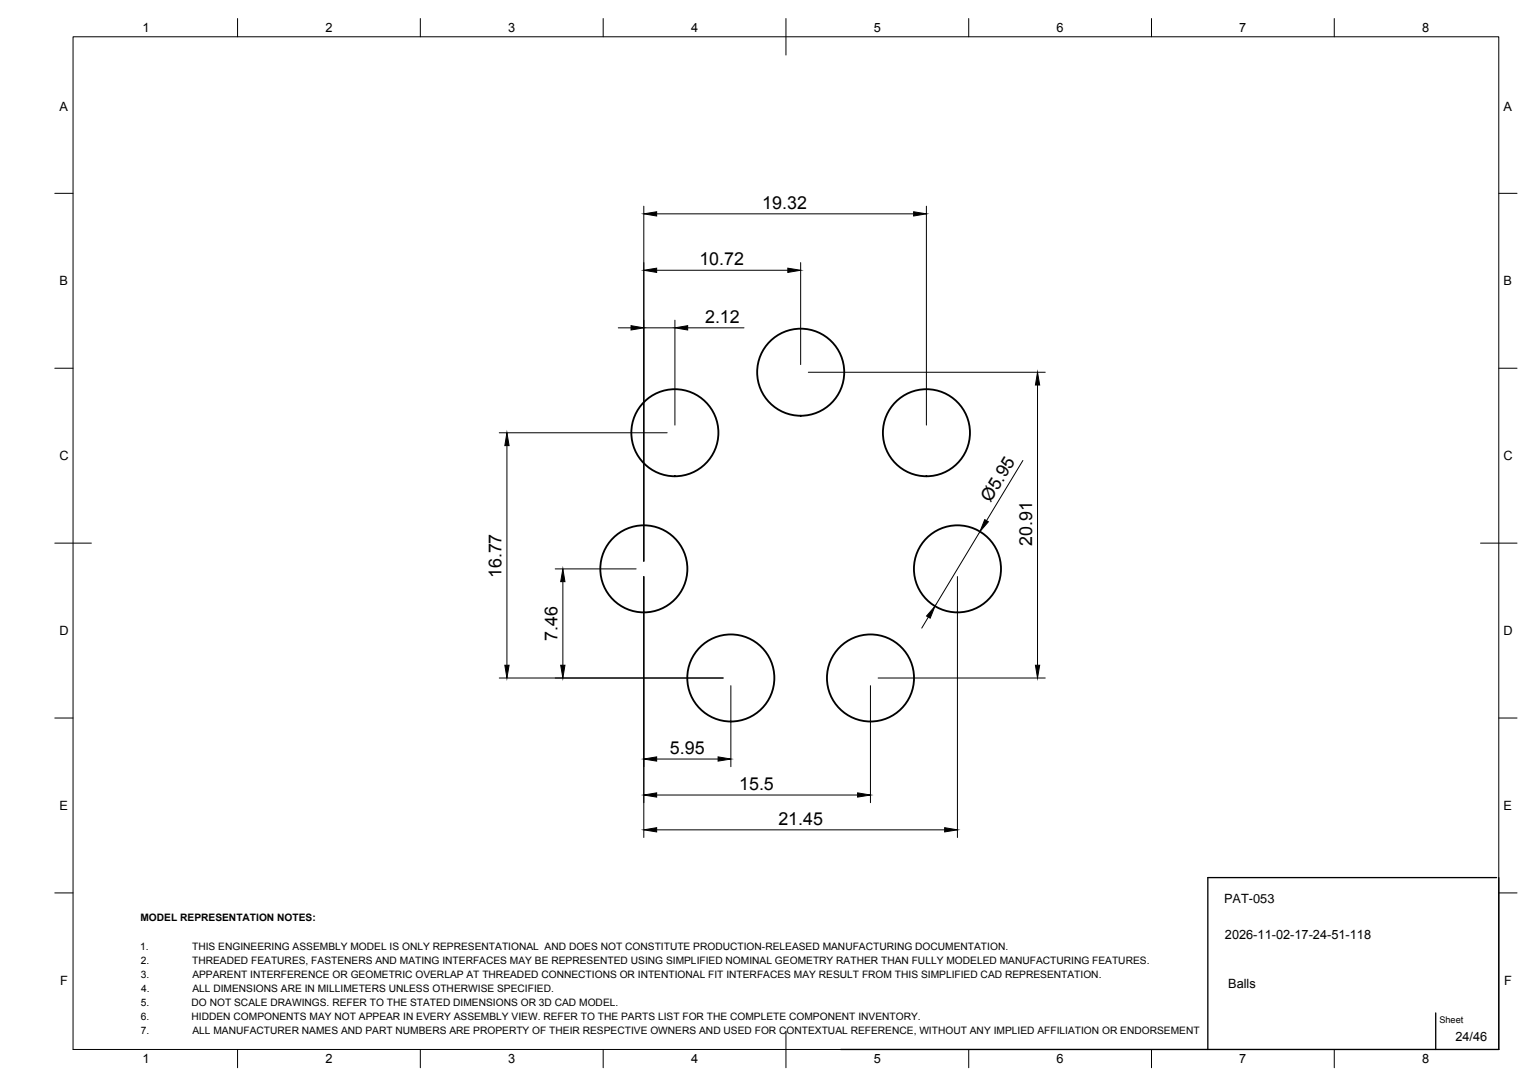
ISO-10303-21;
HEADER;
/* Generated by software containing ST-Developer
 * from STEP Tools, Inc. (www.steptools.com) 
 */

FILE_DESCRIPTION(
/* description */ ('Hand-operated arbor press'),
/* implementation_level */ '2;1');

FILE_NAME(
/* name */ 'Balls.step',
/* time_stamp */ '2026-10-28T03:25:25-07:00',
/* author */ (''),
/* organization */ (''),
/* preprocessor_version */ 'ST-DEVELOPER v20.2',
/* originating_system */ 'Autodesk Translation Framework v15.17.0.0',
/* authorisation */ '');

FILE_SCHEMA (('AUTOMOTIVE_DESIGN { 1 0 10303 214 3 1 1 }'));
ENDSEC;

DATA;
#10=MECHANICAL_DESIGN_GEOMETRIC_PRESENTATION_REPRESENTATION('',(#604,#605,#606,#607,#608,#609,#610),#32751);
#457=SPHERICAL_SURFACE('',#13456,0.29765);
#458=SPHERICAL_SURFACE('',#13458,0.29765);
#459=SPHERICAL_SURFACE('',#13460,0.29765);
#460=SPHERICAL_SURFACE('',#13462,0.29765);
#461=SPHERICAL_SURFACE('',#13464,0.29765);
#462=SPHERICAL_SURFACE('',#13466,0.29765);
#463=SPHERICAL_SURFACE('',#13468,0.29765);
#520=SHAPE_REPRESENTATION_RELATIONSHIP('SRR','None',#32950,#562);
#562=ADVANCED_BREP_SHAPE_REPRESENTATION('',(#652,#653,#654,#655,#656,#657,
#658),#32724);
#604=STYLED_ITEM('',(#33242),#652);
#605=STYLED_ITEM('',(#33242),#653);
#606=STYLED_ITEM('',(#33242),#654);
#607=STYLED_ITEM('',(#33242),#655);
#608=STYLED_ITEM('',(#33242),#656);
#609=STYLED_ITEM('',(#33242),#657);
#610=STYLED_ITEM('',(#33242),#658);
#652=MANIFOLD_SOLID_BREP('Body1',#12502);
#653=MANIFOLD_SOLID_BREP('Body2',#12503);
#654=MANIFOLD_SOLID_BREP('Body3',#12504);
#655=MANIFOLD_SOLID_BREP('Body4',#12505);
#656=MANIFOLD_SOLID_BREP('Body5',#12506);
#657=MANIFOLD_SOLID_BREP('Body6',#12507);
#658=MANIFOLD_SOLID_BREP('Body7',#12508);
#1528=FACE_OUTER_BOUND('',#2335,.T.);
#1529=FACE_OUTER_BOUND('',#2336,.T.);
#1530=FACE_OUTER_BOUND('',#2337,.T.);
#1531=FACE_OUTER_BOUND('',#2338,.T.);
#1532=FACE_OUTER_BOUND('',#2339,.T.);
#1533=FACE_OUTER_BOUND('',#2340,.T.);
#1534=FACE_OUTER_BOUND('',#2341,.T.);
#2335=EDGE_LOOP('',(#9406,#9407));
#2336=EDGE_LOOP('',(#9408,#9409));
#2337=EDGE_LOOP('',(#9410,#9411));
#2338=EDGE_LOOP('',(#9412,#9413));
#2339=EDGE_LOOP('',(#9414,#9415));
#2340=EDGE_LOOP('',(#9416,#9417));
#2341=EDGE_LOOP('',(#9418,#9419));
#5366=CIRCLE('',#13457,0.29765);
#5367=CIRCLE('',#13459,0.29765);
#5368=CIRCLE('',#13461,0.29765);
#5369=CIRCLE('',#13463,0.29765);
#5370=CIRCLE('',#13465,0.29765);
#5371=CIRCLE('',#13467,0.29765);
#5372=CIRCLE('',#13469,0.29765);
#5914=VERTEX_POINT('',#18795);
#5915=VERTEX_POINT('',#18796);
#5916=VERTEX_POINT('',#18799);
#5917=VERTEX_POINT('',#18800);
#5918=VERTEX_POINT('',#18803);
#5919=VERTEX_POINT('',#18804);
#5920=VERTEX_POINT('',#18807);
#5921=VERTEX_POINT('',#18808);
#5922=VERTEX_POINT('',#18811);
#5923=VERTEX_POINT('',#18812);
#5924=VERTEX_POINT('',#18815);
#5925=VERTEX_POINT('',#18816);
#5926=VERTEX_POINT('',#18819);
#5927=VERTEX_POINT('',#18820);
#7206=EDGE_CURVE('',#5914,#5915,#5366,.T.);
#7207=EDGE_CURVE('',#5916,#5917,#5367,.T.);
#7208=EDGE_CURVE('',#5918,#5919,#5368,.T.);
#7209=EDGE_CURVE('',#5920,#5921,#5369,.T.);
#7210=EDGE_CURVE('',#5922,#5923,#5370,.T.);
#7211=EDGE_CURVE('',#5924,#5925,#5371,.T.);
#7212=EDGE_CURVE('',#5926,#5927,#5372,.T.);
#9406=ORIENTED_EDGE('',*,*,#7206,.T.);
#9407=ORIENTED_EDGE('',*,*,#7206,.F.);
#9408=ORIENTED_EDGE('',*,*,#7207,.T.);
#9409=ORIENTED_EDGE('',*,*,#7207,.F.);
#9410=ORIENTED_EDGE('',*,*,#7208,.T.);
#9411=ORIENTED_EDGE('',*,*,#7208,.F.);
#9412=ORIENTED_EDGE('',*,*,#7209,.T.);
#9413=ORIENTED_EDGE('',*,*,#7209,.F.);
#9414=ORIENTED_EDGE('',*,*,#7210,.T.);
#9415=ORIENTED_EDGE('',*,*,#7210,.F.);
#9416=ORIENTED_EDGE('',*,*,#7211,.T.);
#9417=ORIENTED_EDGE('',*,*,#7211,.F.);
#9418=ORIENTED_EDGE('',*,*,#7212,.T.);
#9419=ORIENTED_EDGE('',*,*,#7212,.F.);
#12037=ADVANCED_FACE('',(#1528),#457,.T.);
#12038=ADVANCED_FACE('',(#1529),#458,.T.);
#12039=ADVANCED_FACE('',(#1530),#459,.T.);
#12040=ADVANCED_FACE('',(#1531),#460,.T.);
#12041=ADVANCED_FACE('',(#1532),#461,.T.);
#12042=ADVANCED_FACE('',(#1533),#462,.T.);
#12043=ADVANCED_FACE('',(#1534),#463,.T.);
#12502=CLOSED_SHELL('',(#12037));
#12503=CLOSED_SHELL('',(#12038));
#12504=CLOSED_SHELL('',(#12039));
#12505=CLOSED_SHELL('',(#12040));
#12506=CLOSED_SHELL('',(#12041));
#12507=CLOSED_SHELL('',(#12042));
#12508=CLOSED_SHELL('',(#12043));
#13455=AXIS2_PLACEMENT_3D('',#18793,#15408,#15409);
#13456=AXIS2_PLACEMENT_3D('',#18794,#15410,#15411);
#13457=AXIS2_PLACEMENT_3D('',#18797,#15412,#15413);
#13458=AXIS2_PLACEMENT_3D('',#18798,#15414,#15415);
#13459=AXIS2_PLACEMENT_3D('',#18801,#15416,#15417);
#13460=AXIS2_PLACEMENT_3D('',#18802,#15418,#15419);
#13461=AXIS2_PLACEMENT_3D('',#18805,#15420,#15421);
#13462=AXIS2_PLACEMENT_3D('',#18806,#15422,#15423);
#13463=AXIS2_PLACEMENT_3D('',#18809,#15424,#15425);
#13464=AXIS2_PLACEMENT_3D('',#18810,#15426,#15427);
#13465=AXIS2_PLACEMENT_3D('',#18813,#15428,#15429);
#13466=AXIS2_PLACEMENT_3D('',#18814,#15430,#15431);
#13467=AXIS2_PLACEMENT_3D('',#18817,#15432,#15433);
#13468=AXIS2_PLACEMENT_3D('',#18818,#15434,#15435);
#13469=AXIS2_PLACEMENT_3D('',#18821,#15436,#15437);
#15408=DIRECTION('axis',(0.,0.,1.));
#15409=DIRECTION('refdir',(1.,0.,0.));
#15410=DIRECTION('center_axis',(0.,0.,1.));
#15411=DIRECTION('ref_axis',(1.,0.,0.));
#15412=DIRECTION('center_axis',(1.22464679914735E-16,-1.,0.));
#15413=DIRECTION('ref_axis',(-1.,-1.22464679914735E-16,0.));
#15414=DIRECTION('center_axis',(0.78183148246803,0.,0.623489801858733));
#15415=DIRECTION('ref_axis',(0.623489801858734,0.,-0.78183148246803));
#15416=DIRECTION('center_axis',(7.63554790147315E-17,-1.,-9.57467422477103E-17));
#15417=DIRECTION('ref_axis',(-0.623489801858734,-1.22464679914735E-16,0.78183148246803));
#15418=DIRECTION('center_axis',(0.974927912181824,0.,-0.222520933956314));
#15419=DIRECTION('ref_axis',(-0.222520933956314,0.,-0.974927912181824));
#15420=DIRECTION('center_axis',(-2.7250954951288E-17,-1.,-1.19394234705288E-16));
#15421=DIRECTION('ref_axis',(0.222520933956314,-1.22464679914735E-16,0.974927912181824));
#15422=DIRECTION('center_axis',(0.433883739117558,0.,-0.900968867902419));
#15423=DIRECTION('ref_axis',(-0.900968867902419,0.,-0.433883739117558));
#15424=DIRECTION('center_axis',(-1.10336864020811E-16,-1.,-5.31354332312403E-17));
#15425=DIRECTION('ref_axis',(0.900968867902419,-1.22464679914735E-16,0.433883739117558));
#15426=DIRECTION('center_axis',(-0.433883739117558,0.,-0.900968867902419));
#15427=DIRECTION('ref_axis',(-0.900968867902419,0.,0.433883739117558));
#15428=DIRECTION('center_axis',(-1.10336864020811E-16,-1.,5.31354332312403E-17));
#15429=DIRECTION('ref_axis',(0.900968867902419,-1.22464679914735E-16,-0.433883739117558));
#15430=DIRECTION('center_axis',(-0.974927912181824,0.,-0.222520933956314));
#15431=DIRECTION('ref_axis',(-0.222520933956315,0.,0.974927912181824));
#15432=DIRECTION('center_axis',(-2.7250954951288E-17,-1.,1.19394234705288E-16));
#15433=DIRECTION('ref_axis',(0.222520933956315,-1.22464679914735E-16,-0.974927912181824));
#15434=DIRECTION('center_axis',(-0.78183148246803,0.,0.623489801858734));
#15435=DIRECTION('ref_axis',(0.623489801858733,0.,0.78183148246803));
#15436=DIRECTION('center_axis',(7.63554790147315E-17,-1.,9.57467422477103E-17));
#15437=DIRECTION('ref_axis',(-0.623489801858733,-1.22464679914735E-16,-0.78183148246803));
#18793=CARTESIAN_POINT('',(0.,0.,0.));
#18794=CARTESIAN_POINT('Origin',(1.1,0.,0.));
#18795=CARTESIAN_POINT('',(1.1,-2.23201749654651E-33,0.29765));
#18796=CARTESIAN_POINT('',(1.1,-2.23201749654651E-33,-0.29765));
#18797=CARTESIAN_POINT('Origin',(1.1,0.,0.));
#18798=CARTESIAN_POINT('Origin',(0.685838782044607,0.,-0.860014630714833));
#18799=CARTESIAN_POINT('',(0.918550922801216,-5.31350540756609E-33,-0.674432891191581));
#18800=CARTESIAN_POINT('',(0.453126641287998,8.49470414473068E-34,-1.04559637023808));
#18801=CARTESIAN_POINT('Origin',(0.685838782044607,0.,-0.860014630714833));
#18802=CARTESIAN_POINT('Origin',(-0.244773027351946,0.,-1.07242070340001));
#18803=CARTESIAN_POINT('',(0.0454142657089739,-2.23201749654651E-33,-1.1386540593921));
#18804=CARTESIAN_POINT('',(-0.534960320412865,-2.23201749654651E-33,-1.00618734740791));
#18805=CARTESIAN_POINT('Origin',(-0.244773027351946,0.,-1.07242070340001));
#18806=CARTESIAN_POINT('Origin',(-0.991065754692661,0.,-0.477272113029314));
#18807=CARTESIAN_POINT('',(-0.86192025974432,8.49470414473067E-34,-0.745445496560469));
#18808=CARTESIAN_POINT('',(-1.120211249641,-5.31350540756609E-33,-0.209098729498159));
#18809=CARTESIAN_POINT('Origin',(-0.991065754692661,0.,-0.477272113029314));
#18810=CARTESIAN_POINT('Origin',(-0.991065754692661,0.,0.477272113029314));
#18811=CARTESIAN_POINT('',(-1.120211249641,-2.23201749654651E-33,0.209098729498159));
#18812=CARTESIAN_POINT('',(-0.86192025974432,-2.23201749654651E-33,0.745445496560469));
#18813=CARTESIAN_POINT('Origin',(-0.991065754692661,0.,0.477272113029314));
#18814=CARTESIAN_POINT('Origin',(-0.244773027351946,0.,1.07242070340001));
#18815=CARTESIAN_POINT('',(-0.534960320412866,-2.23201749654651E-33,1.00618734740791));
#18816=CARTESIAN_POINT('',(0.0454142657089737,-2.23201749654651E-33,1.1386540593921));
#18817=CARTESIAN_POINT('Origin',(-0.244773027351946,0.,1.07242070340001));
#18818=CARTESIAN_POINT('Origin',(0.685838782044607,0.,0.860014630714833));
#18819=CARTESIAN_POINT('',(0.453126641287998,-2.23201749654651E-33,1.04559637023808));
#18820=CARTESIAN_POINT('',(0.918550922801216,-2.23201749654651E-33,0.674432891191581));
#18821=CARTESIAN_POINT('Origin',(0.685838782044607,0.,0.860014630714833));
#32675=UNCERTAINTY_MEASURE_WITH_UNIT(LENGTH_MEASURE(0.001),#32752,
'DISTANCE_ACCURACY_VALUE',
'Maximum model space distance between geometric entities at asserted c
onnectivities');
#32702=UNCERTAINTY_MEASURE_WITH_UNIT(LENGTH_MEASURE(0.001),#32752,
'DISTANCE_ACCURACY_VALUE',
'Maximum model space distance between geometric entities at asserted c
onnectivities');
#32724=(
GEOMETRIC_REPRESENTATION_CONTEXT(3)
GLOBAL_UNCERTAINTY_ASSIGNED_CONTEXT((#32675))
GLOBAL_UNIT_ASSIGNED_CONTEXT((#32752,#32754,#32755))
REPRESENTATION_CONTEXT('','3D')
);
#32751=(
GEOMETRIC_REPRESENTATION_CONTEXT(3)
GLOBAL_UNCERTAINTY_ASSIGNED_CONTEXT((#32702))
GLOBAL_UNIT_ASSIGNED_CONTEXT((#32752,#32754,#32755))
REPRESENTATION_CONTEXT('','3D')
);
#32752=(
LENGTH_UNIT()
NAMED_UNIT(*)
SI_UNIT(.CENTI.,.METRE.)
);
#32754=(
NAMED_UNIT(*)
PLANE_ANGLE_UNIT()
SI_UNIT($,.RADIAN.)
);
#32755=(
NAMED_UNIT(*)
SI_UNIT($,.STERADIAN.)
SOLID_ANGLE_UNIT()
);
#32777=SHAPE_DEFINITION_REPRESENTATION(#32825,#32950);
#32825=PRODUCT_DEFINITION_SHAPE('',$,#32999);
#32950=SHAPE_REPRESENTATION('',(#13455),#32724);
#32977=PRODUCT_DEFINITION_CONTEXT('part definition',#33123,'design');
#32999=PRODUCT_DEFINITION('Balls','Balls',#33047,#32977);
#33047=PRODUCT_DEFINITION_FORMATION('',$,#33146);
#33123=APPLICATION_CONTEXT(
'Core Data for Automotive Mechanical Design Process');
#33124=PRODUCT_CONTEXT('part definition',#33123,'mechanical');
#33146=PRODUCT('Balls','Balls','Balls',(#33124));
#33236=COLOUR_RGB('Grey',0.48,0.52,0.57);
#33237=FILL_AREA_STYLE_COLOUR('',#33236);
#33238=FILL_AREA_STYLE('',(#33237));
#33239=SURFACE_STYLE_FILL_AREA(#33238);
#33240=SURFACE_SIDE_STYLE('',(#33239));
#33241=SURFACE_STYLE_USAGE(.BOTH.,#33240);
#33242=PRESENTATION_STYLE_ASSIGNMENT((#33241));
ENDSEC;
END-ISO-10303-21;
